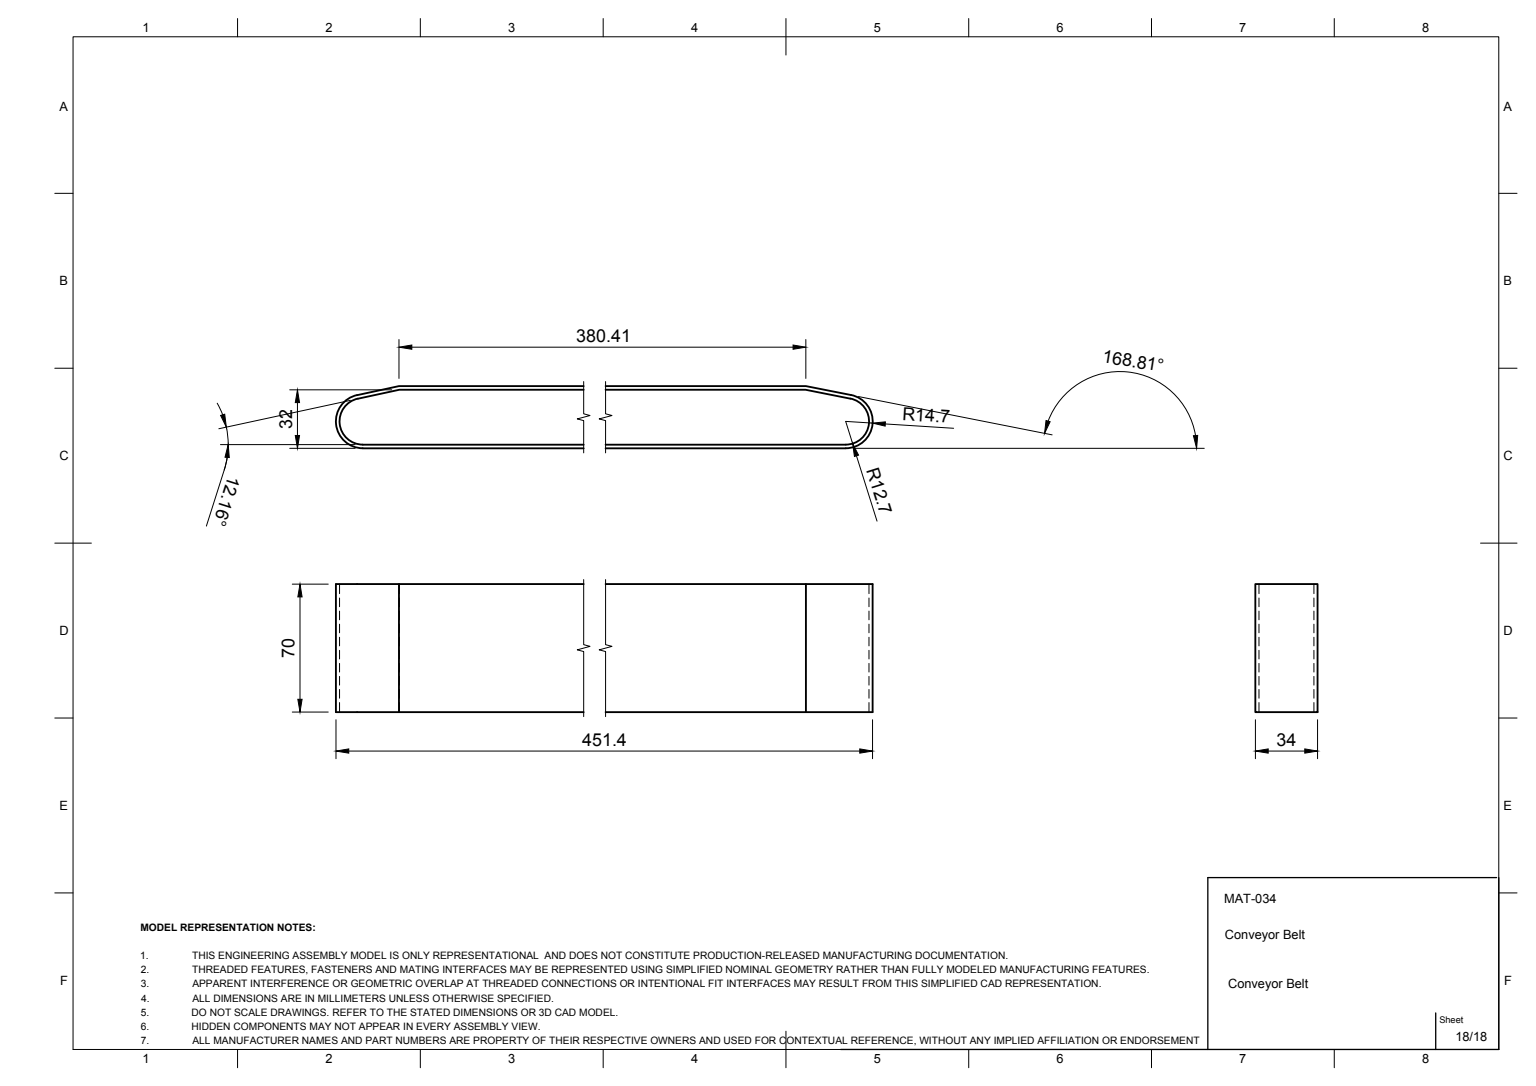
ISO-10303-21;
HEADER;
/* Generated by software containing ST-Developer
 * from STEP Tools, Inc. (www.steptools.com) 
 */

FILE_DESCRIPTION(
/* description */ ('STEP AP214'),
/* implementation_level */ '2;1');

FILE_NAME(
/* name */ 'Conveyor Belt.step',
/* time_stamp */ '2026-11-14T09:24:36-08:00',
/* author */ (''),
/* organization */ (''),
/* preprocessor_version */ 'ST-DEVELOPER v20.2',
/* originating_system */ 'Autodesk Translation Framework v15.17.0.0',
/* authorisation */ '');

FILE_SCHEMA (('AUTOMOTIVE_DESIGN { 1 0 10303 214 3 1 1 }'));
ENDSEC;

DATA;
#10=MECHANICAL_DESIGN_GEOMETRIC_PRESENTATION_REPRESENTATION('',(#212),#18867);
#180=SHAPE_REPRESENTATION_RELATIONSHIP('SRR','None',#18944,#196);
#196=ADVANCED_BREP_SHAPE_REPRESENTATION('',(#236),#18860);
#212=STYLED_ITEM('',(#19028),#236);
#236=MANIFOLD_SOLID_BREP('Body1',#10967);
#344=FACE_BOUND('',#1704,.T.);
#345=FACE_BOUND('',#1706,.T.);
#558=PLANE('',#11696);
#559=PLANE('',#11699);
#560=PLANE('',#11702);
#561=PLANE('',#11703);
#562=PLANE('',#11704);
#563=PLANE('',#11706);
#564=PLANE('',#11707);
#565=PLANE('',#11708);
#566=PLANE('',#11709);
#567=PLANE('',#11711);
#1012=FACE_OUTER_BOUND('',#1701,.T.);
#1013=FACE_OUTER_BOUND('',#1702,.T.);
#1014=FACE_OUTER_BOUND('',#1703,.T.);
#1015=FACE_OUTER_BOUND('',#1705,.T.);
#1016=FACE_OUTER_BOUND('',#1707,.T.);
#1017=FACE_OUTER_BOUND('',#1708,.T.);
#1018=FACE_OUTER_BOUND('',#1709,.T.);
#1019=FACE_OUTER_BOUND('',#1710,.T.);
#1020=FACE_OUTER_BOUND('',#1711,.T.);
#1021=FACE_OUTER_BOUND('',#1712,.T.);
#1022=FACE_OUTER_BOUND('',#1713,.T.);
#1023=FACE_OUTER_BOUND('',#1714,.T.);
#1024=FACE_OUTER_BOUND('',#1715,.T.);
#1025=FACE_OUTER_BOUND('',#1716,.T.);
#1701=EDGE_LOOP('',(#8508,#8509,#8510,#8511));
#1702=EDGE_LOOP('',(#8512,#8513,#8514,#8515));
#1703=EDGE_LOOP('',(#8516,#8517,#8518,#8519,#8520,#8521));
#1704=EDGE_LOOP('',(#8522,#8523,#8524,#8525,#8526,#8527));
#1705=EDGE_LOOP('',(#8528,#8529,#8530,#8531,#8532,#8533));
#1706=EDGE_LOOP('',(#8534,#8535,#8536,#8537,#8538,#8539));
#1707=EDGE_LOOP('',(#8540,#8541,#8542,#8543));
#1708=EDGE_LOOP('',(#8544,#8545,#8546,#8547));
#1709=EDGE_LOOP('',(#8548,#8549,#8550,#8551));
#1710=EDGE_LOOP('',(#8552,#8553,#8554,#8555));
#1711=EDGE_LOOP('',(#8556,#8557,#8558,#8559));
#1712=EDGE_LOOP('',(#8560,#8561,#8562,#8563));
#1713=EDGE_LOOP('',(#8564,#8565,#8566,#8567));
#1714=EDGE_LOOP('',(#8568,#8569,#8570,#8571));
#1715=EDGE_LOOP('',(#8572,#8573,#8574,#8575));
#1716=EDGE_LOOP('',(#8576,#8577,#8578,#8579));
#2510=LINE('',#17122,#3524);
#2511=LINE('',#17125,#3525);
#2512=LINE('',#17131,#3526);
#2513=LINE('',#17134,#3527);
#2514=LINE('',#17137,#3528);
#2515=LINE('',#17139,#3529);
#2516=LINE('',#17141,#3530);
#2517=LINE('',#17144,#3531);
#2518=LINE('',#17146,#3532);
#2519=LINE('',#17148,#3533);
#2520=LINE('',#17152,#3534);
#2521=LINE('',#17153,#3535);
#2522=LINE('',#17156,#3536);
#2523=LINE('',#17160,#3537);
#2524=LINE('',#17162,#3538);
#2525=LINE('',#17163,#3539);
#2526=LINE('',#17165,#3540);
#2527=LINE('',#17167,#3541);
#2528=LINE('',#17169,#3542);
#2529=LINE('',#17172,#3543);
#2530=LINE('',#17174,#3544);
#2531=LINE('',#17176,#3545);
#2532=LINE('',#17178,#3546);
#2533=LINE('',#17180,#3547);
#2534=LINE('',#17183,#3548);
#2535=LINE('',#17185,#3549);
#2536=LINE('',#17187,#3550);
#2537=LINE('',#17189,#3551);
#3524=VECTOR('',#13832,1000.);
#3525=VECTOR('',#13835,1000.);
#3526=VECTOR('',#13840,1000.);
#3527=VECTOR('',#13843,1000.);
#3528=VECTOR('',#13846,1000.);
#3529=VECTOR('',#13847,1000.);
#3530=VECTOR('',#13848,1000.);
#3531=VECTOR('',#13851,1000.);
#3532=VECTOR('',#13852,1000.);
#3533=VECTOR('',#13853,1000.);
#3534=VECTOR('',#13856,1000.);
#3535=VECTOR('',#13857,1000.);
#3536=VECTOR('',#13860,1000.);
#3537=VECTOR('',#13863,1000.);
#3538=VECTOR('',#13864,1000.);
#3539=VECTOR('',#13865,1000.);
#3540=VECTOR('',#13866,1000.);
#3541=VECTOR('',#13867,1000.);
#3542=VECTOR('',#13868,1000.);
#3543=VECTOR('',#13871,1000.);
#3544=VECTOR('',#13874,1000.);
#3545=VECTOR('',#13877,1000.);
#3546=VECTOR('',#13880,1000.);
#3547=VECTOR('',#13883,1000.);
#3548=VECTOR('',#13888,1000.);
#3549=VECTOR('',#13891,1000.);
#3550=VECTOR('',#13894,1000.);
#3551=VECTOR('',#13897,1000.);
#4304=CIRCLE('',#11691,12.7);
#4305=CIRCLE('',#11692,12.7);
#4306=CIRCLE('',#11694,14.7);
#4307=CIRCLE('',#11695,14.7);
#4308=CIRCLE('',#11697,14.7);
#4309=CIRCLE('',#11698,12.7);
#4310=CIRCLE('',#11700,14.7);
#4311=CIRCLE('',#11701,12.7);
#5036=VERTEX_POINT('',#17118);
#5037=VERTEX_POINT('',#17119);
#5038=VERTEX_POINT('',#17121);
#5039=VERTEX_POINT('',#17123);
#5040=VERTEX_POINT('',#17127);
#5041=VERTEX_POINT('',#17128);
#5042=VERTEX_POINT('',#17130);
#5043=VERTEX_POINT('',#17132);
#5044=VERTEX_POINT('',#17136);
#5045=VERTEX_POINT('',#17138);
#5046=VERTEX_POINT('',#17140);
#5047=VERTEX_POINT('',#17142);
#5048=VERTEX_POINT('',#17145);
#5049=VERTEX_POINT('',#17147);
#5050=VERTEX_POINT('',#17149);
#5051=VERTEX_POINT('',#17151);
#5052=VERTEX_POINT('',#17155);
#5053=VERTEX_POINT('',#17157);
#5054=VERTEX_POINT('',#17159);
#5055=VERTEX_POINT('',#17161);
#5056=VERTEX_POINT('',#17164);
#5057=VERTEX_POINT('',#17166);
#5058=VERTEX_POINT('',#17168);
#5059=VERTEX_POINT('',#17170);
#6287=EDGE_CURVE('',#5036,#5037,#4304,.T.);
#6288=EDGE_CURVE('',#5037,#5038,#2510,.T.);
#6289=EDGE_CURVE('',#5039,#5038,#4305,.T.);
#6290=EDGE_CURVE('',#5036,#5039,#2511,.T.);
#6291=EDGE_CURVE('',#5040,#5041,#4306,.T.);
#6292=EDGE_CURVE('',#5040,#5042,#2512,.T.);
#6293=EDGE_CURVE('',#5042,#5043,#4307,.T.);
#6294=EDGE_CURVE('',#5041,#5043,#2513,.T.);
#6295=EDGE_CURVE('',#5041,#5044,#2514,.T.);
#6296=EDGE_CURVE('',#5044,#5045,#2515,.T.);
#6297=EDGE_CURVE('',#5045,#5046,#2516,.T.);
#6298=EDGE_CURVE('',#5046,#5047,#4308,.T.);
#6299=EDGE_CURVE('',#5047,#5040,#2517,.T.);
#6300=EDGE_CURVE('',#5037,#5048,#2518,.T.);
#6301=EDGE_CURVE('',#5049,#5036,#2519,.T.);
#6302=EDGE_CURVE('',#5050,#5049,#4309,.T.);
#6303=EDGE_CURVE('',#5051,#5050,#2520,.T.);
#6304=EDGE_CURVE('',#5048,#5051,#2521,.T.);
#6305=EDGE_CURVE('',#5052,#5042,#2522,.T.);
#6306=EDGE_CURVE('',#5053,#5052,#4310,.T.);
#6307=EDGE_CURVE('',#5054,#5053,#2523,.T.);
#6308=EDGE_CURVE('',#5055,#5054,#2524,.T.);
#6309=EDGE_CURVE('',#5043,#5055,#2525,.T.);
#6310=EDGE_CURVE('',#5038,#5056,#2526,.T.);
#6311=EDGE_CURVE('',#5056,#5057,#2527,.T.);
#6312=EDGE_CURVE('',#5057,#5058,#2528,.T.);
#6313=EDGE_CURVE('',#5058,#5059,#4311,.T.);
#6314=EDGE_CURVE('',#5059,#5039,#2529,.T.);
#6315=EDGE_CURVE('',#5044,#5055,#2530,.T.);
#6316=EDGE_CURVE('',#5045,#5054,#2531,.T.);
#6317=EDGE_CURVE('',#5046,#5053,#2532,.T.);
#6318=EDGE_CURVE('',#5047,#5052,#2533,.T.);
#6319=EDGE_CURVE('',#5048,#5056,#2534,.T.);
#6320=EDGE_CURVE('',#5051,#5057,#2535,.T.);
#6321=EDGE_CURVE('',#5050,#5058,#2536,.T.);
#6322=EDGE_CURVE('',#5049,#5059,#2537,.T.);
#8508=ORIENTED_EDGE('',*,*,#6287,.T.);
#8509=ORIENTED_EDGE('',*,*,#6288,.T.);
#8510=ORIENTED_EDGE('',*,*,#6289,.F.);
#8511=ORIENTED_EDGE('',*,*,#6290,.F.);
#8512=ORIENTED_EDGE('',*,*,#6291,.F.);
#8513=ORIENTED_EDGE('',*,*,#6292,.T.);
#8514=ORIENTED_EDGE('',*,*,#6293,.T.);
#8515=ORIENTED_EDGE('',*,*,#6294,.F.);
#8516=ORIENTED_EDGE('',*,*,#6291,.T.);
#8517=ORIENTED_EDGE('',*,*,#6295,.T.);
#8518=ORIENTED_EDGE('',*,*,#6296,.T.);
#8519=ORIENTED_EDGE('',*,*,#6297,.T.);
#8520=ORIENTED_EDGE('',*,*,#6298,.T.);
#8521=ORIENTED_EDGE('',*,*,#6299,.T.);
#8522=ORIENTED_EDGE('',*,*,#6300,.F.);
#8523=ORIENTED_EDGE('',*,*,#6287,.F.);
#8524=ORIENTED_EDGE('',*,*,#6301,.F.);
#8525=ORIENTED_EDGE('',*,*,#6302,.F.);
#8526=ORIENTED_EDGE('',*,*,#6303,.F.);
#8527=ORIENTED_EDGE('',*,*,#6304,.F.);
#8528=ORIENTED_EDGE('',*,*,#6293,.F.);
#8529=ORIENTED_EDGE('',*,*,#6305,.F.);
#8530=ORIENTED_EDGE('',*,*,#6306,.F.);
#8531=ORIENTED_EDGE('',*,*,#6307,.F.);
#8532=ORIENTED_EDGE('',*,*,#6308,.F.);
#8533=ORIENTED_EDGE('',*,*,#6309,.F.);
#8534=ORIENTED_EDGE('',*,*,#6289,.T.);
#8535=ORIENTED_EDGE('',*,*,#6310,.T.);
#8536=ORIENTED_EDGE('',*,*,#6311,.T.);
#8537=ORIENTED_EDGE('',*,*,#6312,.T.);
#8538=ORIENTED_EDGE('',*,*,#6313,.T.);
#8539=ORIENTED_EDGE('',*,*,#6314,.T.);
#8540=ORIENTED_EDGE('',*,*,#6309,.T.);
#8541=ORIENTED_EDGE('',*,*,#6315,.F.);
#8542=ORIENTED_EDGE('',*,*,#6295,.F.);
#8543=ORIENTED_EDGE('',*,*,#6294,.T.);
#8544=ORIENTED_EDGE('',*,*,#6308,.T.);
#8545=ORIENTED_EDGE('',*,*,#6316,.F.);
#8546=ORIENTED_EDGE('',*,*,#6296,.F.);
#8547=ORIENTED_EDGE('',*,*,#6315,.T.);
#8548=ORIENTED_EDGE('',*,*,#6307,.T.);
#8549=ORIENTED_EDGE('',*,*,#6317,.F.);
#8550=ORIENTED_EDGE('',*,*,#6297,.F.);
#8551=ORIENTED_EDGE('',*,*,#6316,.T.);
#8552=ORIENTED_EDGE('',*,*,#6306,.T.);
#8553=ORIENTED_EDGE('',*,*,#6318,.F.);
#8554=ORIENTED_EDGE('',*,*,#6298,.F.);
#8555=ORIENTED_EDGE('',*,*,#6317,.T.);
#8556=ORIENTED_EDGE('',*,*,#6305,.T.);
#8557=ORIENTED_EDGE('',*,*,#6292,.F.);
#8558=ORIENTED_EDGE('',*,*,#6299,.F.);
#8559=ORIENTED_EDGE('',*,*,#6318,.T.);
#8560=ORIENTED_EDGE('',*,*,#6310,.F.);
#8561=ORIENTED_EDGE('',*,*,#6288,.F.);
#8562=ORIENTED_EDGE('',*,*,#6300,.T.);
#8563=ORIENTED_EDGE('',*,*,#6319,.T.);
#8564=ORIENTED_EDGE('',*,*,#6311,.F.);
#8565=ORIENTED_EDGE('',*,*,#6319,.F.);
#8566=ORIENTED_EDGE('',*,*,#6304,.T.);
#8567=ORIENTED_EDGE('',*,*,#6320,.T.);
#8568=ORIENTED_EDGE('',*,*,#6312,.F.);
#8569=ORIENTED_EDGE('',*,*,#6320,.F.);
#8570=ORIENTED_EDGE('',*,*,#6303,.T.);
#8571=ORIENTED_EDGE('',*,*,#6321,.T.);
#8572=ORIENTED_EDGE('',*,*,#6313,.F.);
#8573=ORIENTED_EDGE('',*,*,#6321,.F.);
#8574=ORIENTED_EDGE('',*,*,#6302,.T.);
#8575=ORIENTED_EDGE('',*,*,#6322,.T.);
#8576=ORIENTED_EDGE('',*,*,#6314,.F.);
#8577=ORIENTED_EDGE('',*,*,#6322,.F.);
#8578=ORIENTED_EDGE('',*,*,#6301,.T.);
#8579=ORIENTED_EDGE('',*,*,#6290,.T.);
#10249=CYLINDRICAL_SURFACE('',#11690,12.7);
#10250=CYLINDRICAL_SURFACE('',#11693,14.7);
#10251=CYLINDRICAL_SURFACE('',#11705,14.7);
#10252=CYLINDRICAL_SURFACE('',#11710,12.7);
#10649=ADVANCED_FACE('',(#1012),#10249,.F.);
#10650=ADVANCED_FACE('',(#1013),#10250,.T.);
#10651=ADVANCED_FACE('',(#1014,#344),#558,.T.);
#10652=ADVANCED_FACE('',(#1015,#345),#559,.F.);
#10653=ADVANCED_FACE('',(#1016),#560,.F.);
#10654=ADVANCED_FACE('',(#1017),#561,.F.);
#10655=ADVANCED_FACE('',(#1018),#562,.F.);
#10656=ADVANCED_FACE('',(#1019),#10251,.T.);
#10657=ADVANCED_FACE('',(#1020),#563,.F.);
#10658=ADVANCED_FACE('',(#1021),#564,.T.);
#10659=ADVANCED_FACE('',(#1022),#565,.T.);
#10660=ADVANCED_FACE('',(#1023),#566,.T.);
#10661=ADVANCED_FACE('',(#1024),#10252,.F.);
#10662=ADVANCED_FACE('',(#1025),#567,.T.);
#10967=CLOSED_SHELL('',(#10649,#10650,#10651,#10652,#10653,#10654,#10655,
#10656,#10657,#10658,#10659,#10660,#10661,#10662));
#11689=AXIS2_PLACEMENT_3D('',#17116,#13826,#13827);
#11690=AXIS2_PLACEMENT_3D('',#17117,#13828,#13829);
#11691=AXIS2_PLACEMENT_3D('',#17120,#13830,#13831);
#11692=AXIS2_PLACEMENT_3D('',#17124,#13833,#13834);
#11693=AXIS2_PLACEMENT_3D('',#17126,#13836,#13837);
#11694=AXIS2_PLACEMENT_3D('',#17129,#13838,#13839);
#11695=AXIS2_PLACEMENT_3D('',#17133,#13841,#13842);
#11696=AXIS2_PLACEMENT_3D('',#17135,#13844,#13845);
#11697=AXIS2_PLACEMENT_3D('',#17143,#13849,#13850);
#11698=AXIS2_PLACEMENT_3D('',#17150,#13854,#13855);
#11699=AXIS2_PLACEMENT_3D('',#17154,#13858,#13859);
#11700=AXIS2_PLACEMENT_3D('',#17158,#13861,#13862);
#11701=AXIS2_PLACEMENT_3D('',#17171,#13869,#13870);
#11702=AXIS2_PLACEMENT_3D('',#17173,#13872,#13873);
#11703=AXIS2_PLACEMENT_3D('',#17175,#13875,#13876);
#11704=AXIS2_PLACEMENT_3D('',#17177,#13878,#13879);
#11705=AXIS2_PLACEMENT_3D('',#17179,#13881,#13882);
#11706=AXIS2_PLACEMENT_3D('',#17181,#13884,#13885);
#11707=AXIS2_PLACEMENT_3D('',#17182,#13886,#13887);
#11708=AXIS2_PLACEMENT_3D('',#17184,#13889,#13890);
#11709=AXIS2_PLACEMENT_3D('',#17186,#13892,#13893);
#11710=AXIS2_PLACEMENT_3D('',#17188,#13895,#13896);
#11711=AXIS2_PLACEMENT_3D('',#17190,#13898,#13899);
#13826=DIRECTION('axis',(0.,0.,1.));
#13827=DIRECTION('refdir',(1.,0.,0.));
#13828=DIRECTION('center_axis',(0.,0.,-1.));
#13829=DIRECTION('ref_axis',(-1.,0.,0.));
#13830=DIRECTION('center_axis',(0.,0.,1.));
#13831=DIRECTION('ref_axis',(1.,0.,0.));
#13832=DIRECTION('',(0.,0.,-1.));
#13833=DIRECTION('center_axis',(0.,0.,1.));
#13834=DIRECTION('ref_axis',(1.,0.,0.));
#13835=DIRECTION('',(0.,0.,-1.));
#13836=DIRECTION('center_axis',(0.,0.,-1.));
#13837=DIRECTION('ref_axis',(-1.,0.,0.));
#13838=DIRECTION('center_axis',(0.,0.,1.));
#13839=DIRECTION('ref_axis',(1.,0.,0.));
#13840=DIRECTION('',(0.,0.,-1.));
#13841=DIRECTION('center_axis',(0.,0.,1.));
#13842=DIRECTION('ref_axis',(1.,0.,0.));
#13843=DIRECTION('',(0.,0.,-1.));
#13844=DIRECTION('center_axis',(0.,0.,1.));
#13845=DIRECTION('ref_axis',(1.,0.,0.));
#13846=DIRECTION('',(0.977572309327645,-0.210600047568408,0.));
#13847=DIRECTION('',(1.,1.18563999046388E-16,0.));
#13848=DIRECTION('',(0.980975643997698,0.194130847325459,0.));
#13849=DIRECTION('center_axis',(0.,0.,1.));
#13850=DIRECTION('ref_axis',(-1.,0.,0.));
#13851=DIRECTION('',(-1.,-1.23321574121574E-16,0.));
#13852=DIRECTION('',(0.977572309327645,-0.210600047568409,0.));
#13853=DIRECTION('',(-1.,-1.23321574121574E-16,0.));
#13854=DIRECTION('center_axis',(0.,0.,1.));
#13855=DIRECTION('ref_axis',(-1.,0.,0.));
#13856=DIRECTION('',(0.980975643997698,0.194130847325459,0.));
#13857=DIRECTION('',(1.,1.09561482693272E-16,0.));
#13858=DIRECTION('center_axis',(0.,0.,1.));
#13859=DIRECTION('ref_axis',(1.,0.,0.));
#13860=DIRECTION('',(-1.,-1.23321574121574E-16,0.));
#13861=DIRECTION('center_axis',(0.,0.,1.));
#13862=DIRECTION('ref_axis',(-1.,0.,0.));
#13863=DIRECTION('',(0.980975643997698,0.194130847325459,0.));
#13864=DIRECTION('',(1.,1.18563999046388E-16,0.));
#13865=DIRECTION('',(0.977572309327645,-0.210600047568408,0.));
#13866=DIRECTION('',(0.977572309327645,-0.210600047568409,0.));
#13867=DIRECTION('',(1.,1.09561482693272E-16,0.));
#13868=DIRECTION('',(0.980975643997698,0.194130847325459,0.));
#13869=DIRECTION('center_axis',(0.,0.,1.));
#13870=DIRECTION('ref_axis',(-1.,0.,0.));
#13871=DIRECTION('',(-1.,-1.23321574121574E-16,0.));
#13872=DIRECTION('center_axis',(0.210600047568408,0.977572309327645,0.));
#13873=DIRECTION('ref_axis',(-0.977572309327645,0.210600047568408,0.));
#13874=DIRECTION('',(0.,0.,-1.));
#13875=DIRECTION('center_axis',(-1.18563999046388E-16,1.,0.));
#13876=DIRECTION('ref_axis',(-1.,-1.18563999046388E-16,0.));
#13877=DIRECTION('',(0.,0.,-1.));
#13878=DIRECTION('center_axis',(-0.194130847325459,0.980975643997699,0.));
#13879=DIRECTION('ref_axis',(-0.980975643997699,-0.19413084732546,0.));
#13880=DIRECTION('',(0.,0.,-1.));
#13881=DIRECTION('center_axis',(0.,0.,-1.));
#13882=DIRECTION('ref_axis',(0.995232546693912,0.0975303952680951,0.));
#13883=DIRECTION('',(0.,0.,-1.));
#13884=DIRECTION('center_axis',(1.23321574121574E-16,-1.,0.));
#13885=DIRECTION('ref_axis',(1.,1.23321574121574E-16,0.));
#13886=DIRECTION('center_axis',(0.210600047568409,0.977572309327645,0.));
#13887=DIRECTION('ref_axis',(-0.977572309327645,0.210600047568409,0.));
#13888=DIRECTION('',(0.,0.,-1.));
#13889=DIRECTION('center_axis',(-1.09561482693272E-16,1.,0.));
#13890=DIRECTION('ref_axis',(-1.,-1.09561482693272E-16,0.));
#13891=DIRECTION('',(0.,0.,-1.));
#13892=DIRECTION('center_axis',(-0.194130847325459,0.980975643997699,0.));
#13893=DIRECTION('ref_axis',(-0.980975643997699,-0.194130847325459,0.));
#13894=DIRECTION('',(0.,0.,-1.));
#13895=DIRECTION('center_axis',(0.,0.,-1.));
#13896=DIRECTION('ref_axis',(0.995232546693912,0.0975303952680933,0.));
#13897=DIRECTION('',(0.,0.,-1.));
#13898=DIRECTION('center_axis',(1.23321574121574E-16,-1.,0.));
#13899=DIRECTION('ref_axis',(1.,1.23321574121574E-16,0.));
#17116=CARTESIAN_POINT('',(0.,0.,0.));
#17117=CARTESIAN_POINT('Origin',(-211.,0.,35.));
#17118=CARTESIAN_POINT('',(-211.,12.7,35.));
#17119=CARTESIAN_POINT('',(-213.674620604119,-12.4151683284611,35.));
#17120=CARTESIAN_POINT('Origin',(-211.,0.,35.));
#17121=CARTESIAN_POINT('',(-213.674620604119,-12.4151683284611,-35.));
#17122=CARTESIAN_POINT('',(-213.674620604119,-12.4151683284611,35.));
#17123=CARTESIAN_POINT('',(-211.,12.7,-35.));
#17124=CARTESIAN_POINT('Origin',(-211.,0.,-35.));
#17125=CARTESIAN_POINT('',(-211.,12.7,35.));
#17126=CARTESIAN_POINT('Origin',(-211.,0.,35.));
#17127=CARTESIAN_POINT('',(-211.,14.7,35.));
#17128=CARTESIAN_POINT('',(-214.095820699256,-14.3703129471164,35.));
#17129=CARTESIAN_POINT('Origin',(-211.,0.,35.));
#17130=CARTESIAN_POINT('',(-211.,14.7,-35.));
#17131=CARTESIAN_POINT('',(-211.,14.7,35.));
#17132=CARTESIAN_POINT('',(-214.095820699256,-14.3703129471164,-35.));
#17133=CARTESIAN_POINT('Origin',(-211.,0.,-35.));
#17134=CARTESIAN_POINT('',(-214.095820699256,-14.3703129471164,35.));
#17135=CARTESIAN_POINT('Origin',(-211.,0.,35.));
#17136=CARTESIAN_POINT('',(-191.212988467299,-19.2999999999999,35.));
#17137=CARTESIAN_POINT('',(-191.212988467299,-19.2999999999999,35.));
#17138=CARTESIAN_POINT('',(189.195995188445,-19.2999999999999,35.));
#17139=CARTESIAN_POINT('',(189.195995188445,-19.2999999999999,35.));
#17140=CARTESIAN_POINT('',(213.853723455684,-14.4203419667661,35.));
#17141=CARTESIAN_POINT('',(189.195995188445,-19.2999999999999,35.));
#17142=CARTESIAN_POINT('',(211.,14.7000000000001,35.));
#17143=CARTESIAN_POINT('Origin',(211.,5.16800949240183E-14,35.));
#17144=CARTESIAN_POINT('',(-211.,14.7,35.));
#17145=CARTESIAN_POINT('',(-191.,-17.2999999999999,35.));
#17146=CARTESIAN_POINT('',(-191.,-17.2999999999999,35.));
#17147=CARTESIAN_POINT('',(211.,12.7000000000001,35.));
#17148=CARTESIAN_POINT('',(-211.,12.7,35.));
#17149=CARTESIAN_POINT('',(213.465461761033,-12.4583906787707,35.));
#17150=CARTESIAN_POINT('Origin',(211.,5.16800949240183E-14,35.));
#17151=CARTESIAN_POINT('',(189.,-17.2999999999999,35.));
#17152=CARTESIAN_POINT('',(189.,-17.2999999999999,35.));
#17153=CARTESIAN_POINT('',(189.,-17.2999999999999,35.));
#17154=CARTESIAN_POINT('Origin',(-211.,0.,-35.));
#17155=CARTESIAN_POINT('',(211.,14.7000000000001,-35.));
#17156=CARTESIAN_POINT('',(-211.,14.7,-35.));
#17157=CARTESIAN_POINT('',(213.853723455684,-14.4203419667661,-35.));
#17158=CARTESIAN_POINT('Origin',(211.,5.16800949240183E-14,-35.));
#17159=CARTESIAN_POINT('',(189.195995188445,-19.2999999999999,-35.));
#17160=CARTESIAN_POINT('',(189.195995188445,-19.2999999999999,-35.));
#17161=CARTESIAN_POINT('',(-191.212988467299,-19.2999999999999,-35.));
#17162=CARTESIAN_POINT('',(189.195995188445,-19.2999999999999,-35.));
#17163=CARTESIAN_POINT('',(-191.212988467299,-19.2999999999999,-35.));
#17164=CARTESIAN_POINT('',(-191.,-17.2999999999999,-35.));
#17165=CARTESIAN_POINT('',(-191.,-17.2999999999999,-35.));
#17166=CARTESIAN_POINT('',(189.,-17.2999999999999,-35.));
#17167=CARTESIAN_POINT('',(189.,-17.2999999999999,-35.));
#17168=CARTESIAN_POINT('',(213.465461761033,-12.4583906787707,-35.));
#17169=CARTESIAN_POINT('',(189.,-17.2999999999999,-35.));
#17170=CARTESIAN_POINT('',(211.,12.7000000000001,-35.));
#17171=CARTESIAN_POINT('Origin',(211.,5.16800949240183E-14,-35.));
#17172=CARTESIAN_POINT('',(-211.,12.7,-35.));
#17173=CARTESIAN_POINT('Origin',(-191.212988467299,-19.2999999999999,35.));
#17174=CARTESIAN_POINT('',(-191.212988467299,-19.2999999999999,35.));
#17175=CARTESIAN_POINT('Origin',(189.195995188445,-19.2999999999999,35.));
#17176=CARTESIAN_POINT('',(189.195995188445,-19.2999999999999,35.));
#17177=CARTESIAN_POINT('Origin',(189.195995188445,-19.2999999999999,35.));
#17178=CARTESIAN_POINT('',(213.853723455684,-14.4203419667661,35.));
#17179=CARTESIAN_POINT('Origin',(211.,5.16800949240183E-14,35.));
#17180=CARTESIAN_POINT('',(211.,14.7000000000001,35.));
#17181=CARTESIAN_POINT('Origin',(-211.,14.7,35.));
#17182=CARTESIAN_POINT('Origin',(-191.,-17.2999999999999,35.));
#17183=CARTESIAN_POINT('',(-191.,-17.2999999999999,35.));
#17184=CARTESIAN_POINT('Origin',(189.,-17.2999999999999,35.));
#17185=CARTESIAN_POINT('',(189.,-17.2999999999999,35.));
#17186=CARTESIAN_POINT('Origin',(189.,-17.2999999999999,35.));
#17187=CARTESIAN_POINT('',(213.465461761033,-12.4583906787707,35.));
#17188=CARTESIAN_POINT('Origin',(211.,5.16800949240183E-14,35.));
#17189=CARTESIAN_POINT('',(211.,12.7000000000001,35.));
#17190=CARTESIAN_POINT('Origin',(-211.,12.7,35.));
#18842=UNCERTAINTY_MEASURE_WITH_UNIT(LENGTH_MEASURE(0.01),#18868,
'DISTANCE_ACCURACY_VALUE',
'Maximum model space distance between geometric entities at asserted c
onnectivities');
#18849=UNCERTAINTY_MEASURE_WITH_UNIT(LENGTH_MEASURE(0.01),#18868,
'DISTANCE_ACCURACY_VALUE',
'Maximum model space distance between geometric entities at asserted c
onnectivities');
#18860=(
GEOMETRIC_REPRESENTATION_CONTEXT(3)
GLOBAL_UNCERTAINTY_ASSIGNED_CONTEXT((#18842))
GLOBAL_UNIT_ASSIGNED_CONTEXT((#18868,#18870,#18871))
REPRESENTATION_CONTEXT('','3D')
);
#18867=(
GEOMETRIC_REPRESENTATION_CONTEXT(3)
GLOBAL_UNCERTAINTY_ASSIGNED_CONTEXT((#18849))
GLOBAL_UNIT_ASSIGNED_CONTEXT((#18868,#18870,#18871))
REPRESENTATION_CONTEXT('','3D')
);
#18868=(
LENGTH_UNIT()
NAMED_UNIT(*)
SI_UNIT(.MILLI.,.METRE.)
);
#18870=(
NAMED_UNIT(*)
PLANE_ANGLE_UNIT()
SI_UNIT($,.RADIAN.)
);
#18871=(
NAMED_UNIT(*)
SI_UNIT($,.STERADIAN.)
SOLID_ANGLE_UNIT()
);
#18882=SHAPE_DEFINITION_REPRESENTATION(#18899,#18944);
#18899=PRODUCT_DEFINITION_SHAPE('',$,#18962);
#18944=SHAPE_REPRESENTATION('',(#11689),#18860);
#18951=PRODUCT_DEFINITION_CONTEXT('part definition',#19004,'design');
#18962=PRODUCT_DEFINITION('Conveyor Belt','Conveyor Belt',#18979,#18951);
#18979=PRODUCT_DEFINITION_FORMATION('',$,#19016);
#19004=APPLICATION_CONTEXT(
'Core Data for Automotive Mechanical Design Process');
#19005=PRODUCT_CONTEXT('part definition',#19004,'mechanical');
#19016=PRODUCT('Conveyor Belt','Conveyor Belt',$,(#19005));
#19028=PRESENTATION_STYLE_ASSIGNMENT((#19034));
#19034=SURFACE_STYLE_USAGE(.BOTH.,#19040);
#19040=SURFACE_SIDE_STYLE('',(#19046));
#19046=SURFACE_STYLE_FILL_AREA(#19052);
#19052=FILL_AREA_STYLE('Opaque(31,36,43)',(#19058));
#19058=FILL_AREA_STYLE_COLOUR('Opaque(31,36,43)',#19064);
#19064=COLOUR_RGB('Opaque(31,36,43)',0.12156862745098,0.141176470588235,
0.168627450980392);
ENDSEC;
END-ISO-10303-21;
